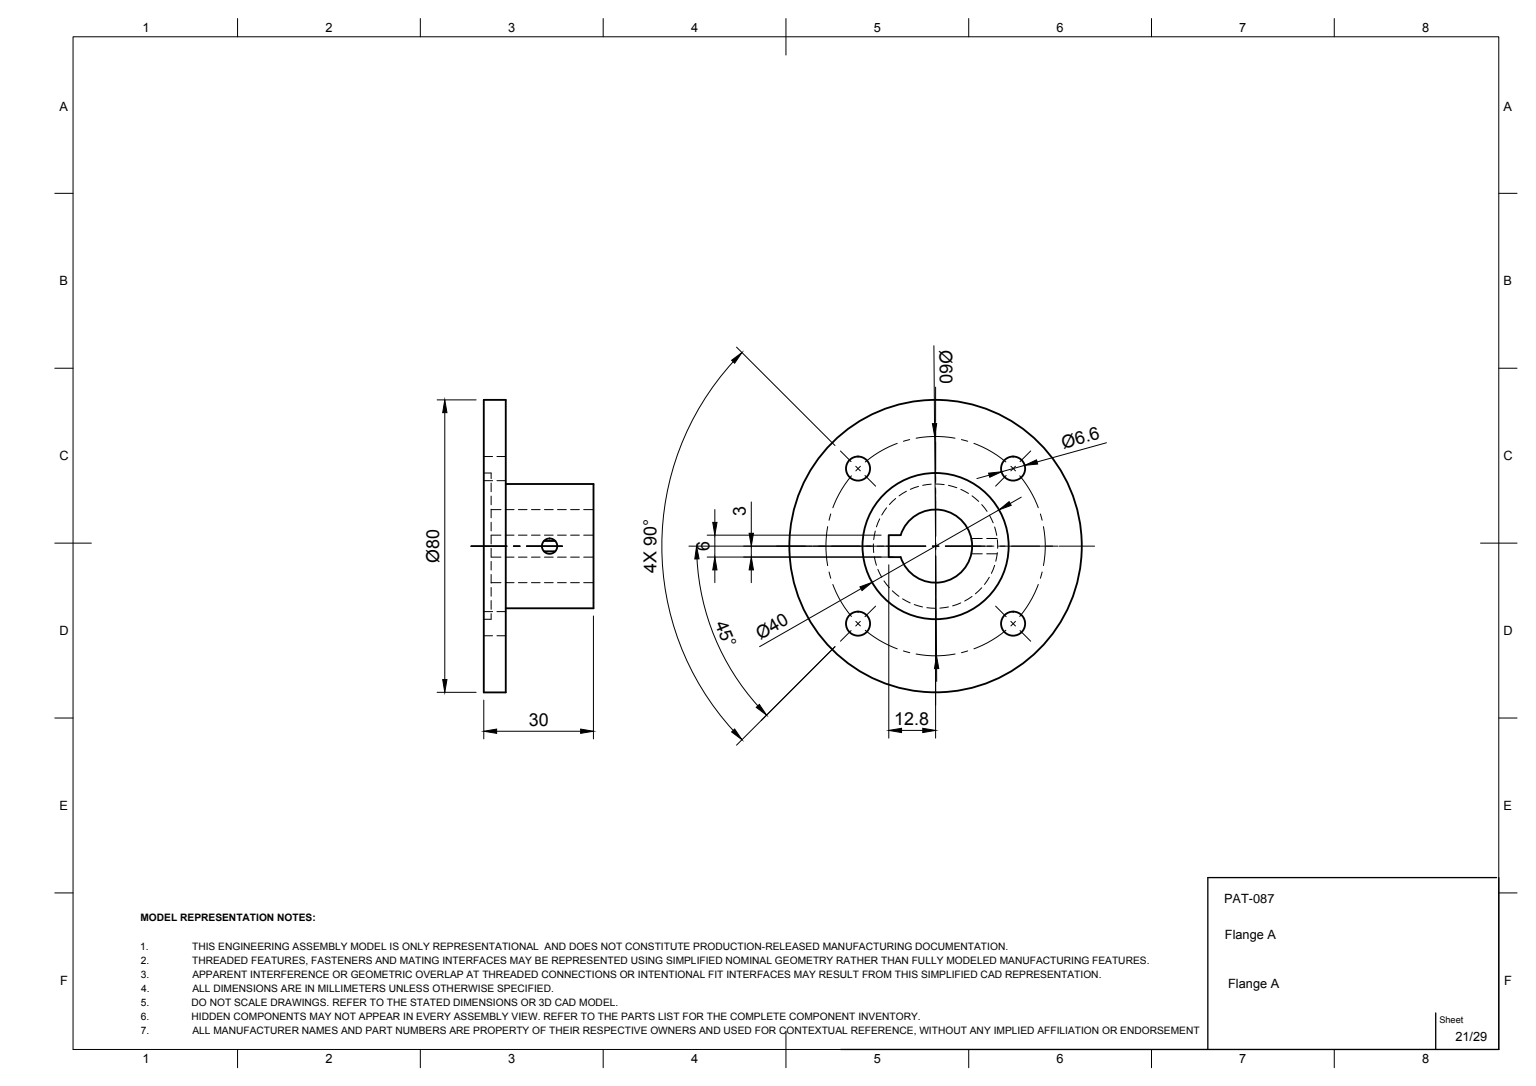
ISO-10303-21;
HEADER;
/* Generated by software containing ST-Developer
 * from STEP Tools, Inc. (www.steptools.com) 
 */

FILE_DESCRIPTION(
/* description */ ('Rigid flange shaft coupling assembly'),
/* implementation_level */ '2;1');

FILE_NAME(
/* name */ 'Flange A.step',
/* time_stamp */ '2026-10-27T10:47:16-07:00',
/* author */ (''),
/* organization */ (''),
/* preprocessor_version */ 'ST-DEVELOPER v20.2',
/* originating_system */ 'Autodesk Translation Framework v15.17.0.0',
/* authorisation */ '');

FILE_SCHEMA (('AUTOMOTIVE_DESIGN { 1 0 10303 214 3 1 1 }'));
ENDSEC;

DATA;
#10=MECHANICAL_DESIGN_GEOMETRIC_PRESENTATION_REPRESENTATION('',(#413),#9141);
#324=B_SPLINE_CURVE_WITH_KNOTS('',3,(#8147,#8148,#8149,#8150,#8151,#8152,
#8153,#8154,#8155,#8156),.UNSPECIFIED.,.F.,.F.,(4,2,2,2,4),(0.803821788694083,
0.87295099185362,0.95230721290097,1.03166343394832,1.10079263710786),
 .UNSPECIFIED.);
#325=B_SPLINE_CURVE_WITH_KNOTS('',3,(#8162,#8163,#8164,#8165,#8166,#8167,
#8168,#8169,#8170,#8171,#8172,#8173,#8174,#8175,#8176,#8177,#8178,#8179),
 .UNSPECIFIED.,.F.,.F.,(4,2,2,2,2,2,2,2,4),(0.,0.0791914196064458,0.158382839212892,
0.237573628052636,0.31676441689238,0.395955205732124,0.475145994571868,
0.554337414178314,0.63352883378476),.UNSPECIFIED.);
#326=B_SPLINE_CURVE_WITH_KNOTS('',3,(#8180,#8181,#8182,#8183,#8184,#8185,
#8186,#8187,#8188,#8189,#8190,#8191,#8192,#8193,#8194,#8195,#8196,#8197),
 .UNSPECIFIED.,.F.,.F.,(4,2,2,2,2,2,2,2,4),(0.63352883378476,0.712720253391205,
0.791911672997651,0.871102461837395,0.95029325067714,1.02948403951688,1.10867482835663,
1.18786624796307,1.26705766756952),.UNSPECIFIED.);
#327=B_SPLINE_CURVE_WITH_KNOTS('',3,(#8200,#8201,#8202,#8203,#8204,#8205,
#8206,#8207,#8208,#8209),.UNSPECIFIED.,.F.,.F.,(4,2,2,2,4),(0.168950313426771,
0.238079516586307,0.317435737633657,0.396791958681006,0.465921161840542),
 .UNSPECIFIED.);
#356=SHAPE_REPRESENTATION_RELATIONSHIP('SRR','None',#9292,#384);
#384=ADVANCED_BREP_SHAPE_REPRESENTATION('',(#441),#9127);
#413=STYLED_ITEM('',(#9493),#441);
#441=MANIFOLD_SOLID_BREP('Body1',#4768);
#519=FACE_BOUND('',#1222,.T.);
#520=FACE_BOUND('',#1225,.T.);
#521=FACE_BOUND('',#1227,.T.);
#522=FACE_BOUND('',#1228,.T.);
#523=FACE_BOUND('',#1229,.T.);
#524=FACE_BOUND('',#1230,.T.);
#525=FACE_BOUND('',#1231,.T.);
#526=FACE_BOUND('',#1234,.T.);
#527=FACE_BOUND('',#1236,.T.);
#528=FACE_BOUND('',#1238,.T.);
#529=FACE_BOUND('',#1239,.T.);
#530=FACE_BOUND('',#1240,.T.);
#531=FACE_BOUND('',#1241,.T.);
#532=FACE_BOUND('',#1242,.T.);
#653=PLANE('',#5338);
#654=PLANE('',#5343);
#655=PLANE('',#5344);
#656=PLANE('',#5345);
#657=PLANE('',#5346);
#658=PLANE('',#5347);
#659=PLANE('',#5353);
#660=PLANE('',#5355);
#661=PLANE('',#5362);
#873=FACE_OUTER_BOUND('',#1211,.T.);
#874=FACE_OUTER_BOUND('',#1212,.T.);
#875=FACE_OUTER_BOUND('',#1213,.T.);
#876=FACE_OUTER_BOUND('',#1214,.T.);
#877=FACE_OUTER_BOUND('',#1215,.T.);
#878=FACE_OUTER_BOUND('',#1216,.T.);
#879=FACE_OUTER_BOUND('',#1217,.T.);
#880=FACE_OUTER_BOUND('',#1218,.T.);
#881=FACE_OUTER_BOUND('',#1219,.T.);
#882=FACE_OUTER_BOUND('',#1220,.T.);
#883=FACE_OUTER_BOUND('',#1221,.T.);
#884=FACE_OUTER_BOUND('',#1223,.T.);
#885=FACE_OUTER_BOUND('',#1224,.T.);
#886=FACE_OUTER_BOUND('',#1226,.T.);
#887=FACE_OUTER_BOUND('',#1232,.T.);
#888=FACE_OUTER_BOUND('',#1233,.T.);
#889=FACE_OUTER_BOUND('',#1235,.T.);
#890=FACE_OUTER_BOUND('',#1237,.T.);
#1211=EDGE_LOOP('',(#3803,#3804,#3805,#3806));
#1212=EDGE_LOOP('',(#3807,#3808,#3809,#3810));
#1213=EDGE_LOOP('',(#3811,#3812,#3813,#3814));
#1214=EDGE_LOOP('',(#3815,#3816,#3817,#3818));
#1215=EDGE_LOOP('',(#3819,#3820));
#1216=EDGE_LOOP('',(#3821,#3822,#3823,#3824,#3825,#3826,#3827,#3828,#3829));
#1217=EDGE_LOOP('',(#3830,#3831,#3832));
#1218=EDGE_LOOP('',(#3833,#3834,#3835,#3836));
#1219=EDGE_LOOP('',(#3837,#3838,#3839,#3840));
#1220=EDGE_LOOP('',(#3841,#3842,#3843,#3844));
#1221=EDGE_LOOP('',(#3845));
#1222=EDGE_LOOP('',(#3846,#3847,#3848,#3849));
#1223=EDGE_LOOP('',(#3850,#3851,#3852,#3853));
#1224=EDGE_LOOP('',(#3854));
#1225=EDGE_LOOP('',(#3855,#3856,#3857,#3858));
#1226=EDGE_LOOP('',(#3859));
#1227=EDGE_LOOP('',(#3860));
#1228=EDGE_LOOP('',(#3861));
#1229=EDGE_LOOP('',(#3862));
#1230=EDGE_LOOP('',(#3863));
#1231=EDGE_LOOP('',(#3864));
#1232=EDGE_LOOP('',(#3865,#3866,#3867,#3868));
#1233=EDGE_LOOP('',(#3869,#3870,#3871,#3872));
#1234=EDGE_LOOP('',(#3873,#3874,#3875,#3876));
#1235=EDGE_LOOP('',(#3877,#3878,#3879,#3880));
#1236=EDGE_LOOP('',(#3881,#3882));
#1237=EDGE_LOOP('',(#3883));
#1238=EDGE_LOOP('',(#3884));
#1239=EDGE_LOOP('',(#3885));
#1240=EDGE_LOOP('',(#3886));
#1241=EDGE_LOOP('',(#3887));
#1242=EDGE_LOOP('',(#3888));
#1578=LINE('',#8120,#1923);
#1579=LINE('',#8126,#1924);
#1580=LINE('',#8132,#1925);
#1581=LINE('',#8138,#1926);
#1582=LINE('',#8143,#1927);
#1583=LINE('',#8160,#1928);
#1584=LINE('',#8211,#1929);
#1585=LINE('',#8215,#1930);
#1586=LINE('',#8217,#1931);
#1587=LINE('',#8219,#1932);
#1588=LINE('',#8220,#1933);
#1589=LINE('',#8223,#1934);
#1590=LINE('',#8225,#1935);
#1591=LINE('',#8226,#1936);
#1592=LINE('',#8229,#1937);
#1593=LINE('',#8231,#1938);
#1594=LINE('',#8232,#1939);
#1595=LINE('',#8241,#1940);
#1596=LINE('',#8253,#1941);
#1597=LINE('',#8256,#1942);
#1923=VECTOR('',#6285,0.33);
#1924=VECTOR('',#6292,0.33);
#1925=VECTOR('',#6299,0.33);
#1926=VECTOR('',#6306,0.33);
#1927=VECTOR('',#6311,1.);
#1928=VECTOR('',#6318,0.21);
#1929=VECTOR('',#6323,1.);
#1930=VECTOR('',#6326,1.);
#1931=VECTOR('',#6327,1.);
#1932=VECTOR('',#6328,1.);
#1933=VECTOR('',#6329,1.);
#1934=VECTOR('',#6332,1.);
#1935=VECTOR('',#6333,1.);
#1936=VECTOR('',#6334,1.);
#1937=VECTOR('',#6337,1.);
#1938=VECTOR('',#6338,1.);
#1939=VECTOR('',#6339,1.);
#1940=VECTOR('',#6350,2.);
#1941=VECTOR('',#6367,4.);
#1942=VECTOR('',#6372,1.7);
#2178=CIRCLE('',#5327,0.33);
#2179=CIRCLE('',#5328,0.33);
#2180=CIRCLE('',#5330,0.33);
#2181=CIRCLE('',#5331,0.33);
#2182=CIRCLE('',#5333,0.33);
#2183=CIRCLE('',#5334,0.33);
#2184=CIRCLE('',#5336,0.33);
#2185=CIRCLE('',#5337,0.33);
#2186=CIRCLE('',#5339,0.21);
#2187=CIRCLE('',#5341,0.21);
#2188=CIRCLE('',#5342,0.21);
#2189=CIRCLE('',#5348,1.7);
#2190=CIRCLE('',#5349,1.);
#2191=CIRCLE('',#5351,2.);
#2192=CIRCLE('',#5352,2.);
#2193=CIRCLE('',#5354,1.);
#2194=CIRCLE('',#5356,4.);
#2195=CIRCLE('',#5357,1.7);
#2196=CIRCLE('',#5359,4.);
#2469=VERTEX_POINT('',#8117);
#2470=VERTEX_POINT('',#8119);
#2471=VERTEX_POINT('',#8123);
#2472=VERTEX_POINT('',#8125);
#2473=VERTEX_POINT('',#8129);
#2474=VERTEX_POINT('',#8131);
#2475=VERTEX_POINT('',#8135);
#2476=VERTEX_POINT('',#8137);
#2477=VERTEX_POINT('',#8141);
#2478=VERTEX_POINT('',#8142);
#2479=VERTEX_POINT('',#8146);
#2480=VERTEX_POINT('',#8157);
#2481=VERTEX_POINT('',#8159);
#2482=VERTEX_POINT('',#8161);
#2483=VERTEX_POINT('',#8198);
#2484=VERTEX_POINT('',#8213);
#2485=VERTEX_POINT('',#8214);
#2486=VERTEX_POINT('',#8216);
#2487=VERTEX_POINT('',#8218);
#2488=VERTEX_POINT('',#8222);
#2489=VERTEX_POINT('',#8224);
#2490=VERTEX_POINT('',#8228);
#2491=VERTEX_POINT('',#8230);
#2492=VERTEX_POINT('',#8234);
#2493=VERTEX_POINT('',#8238);
#2494=VERTEX_POINT('',#8240);
#2495=VERTEX_POINT('',#8246);
#2496=VERTEX_POINT('',#8248);
#2497=VERTEX_POINT('',#8251);
#2945=EDGE_CURVE('',#2469,#2469,#2178,.T.);
#2946=EDGE_CURVE('',#2469,#2470,#1578,.T.);
#2947=EDGE_CURVE('',#2470,#2470,#2179,.T.);
#2948=EDGE_CURVE('',#2471,#2471,#2180,.T.);
#2949=EDGE_CURVE('',#2471,#2472,#1579,.T.);
#2950=EDGE_CURVE('',#2472,#2472,#2181,.T.);
#2951=EDGE_CURVE('',#2473,#2473,#2182,.T.);
#2952=EDGE_CURVE('',#2473,#2474,#1580,.T.);
#2953=EDGE_CURVE('',#2474,#2474,#2183,.T.);
#2954=EDGE_CURVE('',#2475,#2475,#2184,.T.);
#2955=EDGE_CURVE('',#2475,#2476,#1581,.T.);
#2956=EDGE_CURVE('',#2476,#2476,#2185,.T.);
#2957=EDGE_CURVE('',#2477,#2478,#1582,.T.);
#2958=EDGE_CURVE('',#2477,#2478,#2186,.T.);
#2959=EDGE_CURVE('',#2479,#2477,#324,.T.);
#2960=EDGE_CURVE('',#2480,#2479,#2187,.T.);
#2961=EDGE_CURVE('',#2480,#2481,#1583,.T.);
#2962=EDGE_CURVE('',#2482,#2481,#325,.T.);
#2963=EDGE_CURVE('',#2481,#2482,#326,.T.);
#2964=EDGE_CURVE('',#2483,#2480,#2188,.T.);
#2965=EDGE_CURVE('',#2478,#2483,#327,.T.);
#2966=EDGE_CURVE('',#2483,#2479,#1584,.T.);
#2967=EDGE_CURVE('',#2484,#2485,#1585,.T.);
#2968=EDGE_CURVE('',#2484,#2486,#1586,.T.);
#2969=EDGE_CURVE('',#2487,#2486,#1587,.T.);
#2970=EDGE_CURVE('',#2485,#2487,#1588,.T.);
#2971=EDGE_CURVE('',#2488,#2484,#1589,.T.);
#2972=EDGE_CURVE('',#2488,#2489,#1590,.T.);
#2973=EDGE_CURVE('',#2486,#2489,#1591,.T.);
#2974=EDGE_CURVE('',#2490,#2488,#1592,.T.);
#2975=EDGE_CURVE('',#2491,#2490,#1593,.T.);
#2976=EDGE_CURVE('',#2489,#2491,#1594,.T.);
#2977=EDGE_CURVE('',#2492,#2492,#2189,.T.);
#2978=EDGE_CURVE('',#2490,#2485,#2190,.T.);
#2979=EDGE_CURVE('',#2493,#2493,#2191,.T.);
#2980=EDGE_CURVE('',#2493,#2494,#1595,.T.);
#2981=EDGE_CURVE('',#2494,#2494,#2192,.T.);
#2982=EDGE_CURVE('',#2487,#2491,#2193,.T.);
#2983=EDGE_CURVE('',#2495,#2495,#2194,.T.);
#2984=EDGE_CURVE('',#2496,#2496,#2195,.T.);
#2985=EDGE_CURVE('',#2497,#2497,#2196,.T.);
#2986=EDGE_CURVE('',#2497,#2495,#1596,.T.);
#2987=EDGE_CURVE('',#2496,#2492,#1597,.T.);
#3803=ORIENTED_EDGE('',*,*,#2945,.F.);
#3804=ORIENTED_EDGE('',*,*,#2946,.T.);
#3805=ORIENTED_EDGE('',*,*,#2947,.F.);
#3806=ORIENTED_EDGE('',*,*,#2946,.F.);
#3807=ORIENTED_EDGE('',*,*,#2948,.F.);
#3808=ORIENTED_EDGE('',*,*,#2949,.T.);
#3809=ORIENTED_EDGE('',*,*,#2950,.F.);
#3810=ORIENTED_EDGE('',*,*,#2949,.F.);
#3811=ORIENTED_EDGE('',*,*,#2951,.F.);
#3812=ORIENTED_EDGE('',*,*,#2952,.T.);
#3813=ORIENTED_EDGE('',*,*,#2953,.F.);
#3814=ORIENTED_EDGE('',*,*,#2952,.F.);
#3815=ORIENTED_EDGE('',*,*,#2954,.F.);
#3816=ORIENTED_EDGE('',*,*,#2955,.T.);
#3817=ORIENTED_EDGE('',*,*,#2956,.F.);
#3818=ORIENTED_EDGE('',*,*,#2955,.F.);
#3819=ORIENTED_EDGE('',*,*,#2957,.F.);
#3820=ORIENTED_EDGE('',*,*,#2958,.T.);
#3821=ORIENTED_EDGE('',*,*,#2959,.F.);
#3822=ORIENTED_EDGE('',*,*,#2960,.F.);
#3823=ORIENTED_EDGE('',*,*,#2961,.T.);
#3824=ORIENTED_EDGE('',*,*,#2962,.F.);
#3825=ORIENTED_EDGE('',*,*,#2963,.F.);
#3826=ORIENTED_EDGE('',*,*,#2961,.F.);
#3827=ORIENTED_EDGE('',*,*,#2964,.F.);
#3828=ORIENTED_EDGE('',*,*,#2965,.F.);
#3829=ORIENTED_EDGE('',*,*,#2958,.F.);
#3830=ORIENTED_EDGE('',*,*,#2966,.F.);
#3831=ORIENTED_EDGE('',*,*,#2964,.T.);
#3832=ORIENTED_EDGE('',*,*,#2960,.T.);
#3833=ORIENTED_EDGE('',*,*,#2967,.F.);
#3834=ORIENTED_EDGE('',*,*,#2968,.T.);
#3835=ORIENTED_EDGE('',*,*,#2969,.F.);
#3836=ORIENTED_EDGE('',*,*,#2970,.F.);
#3837=ORIENTED_EDGE('',*,*,#2971,.F.);
#3838=ORIENTED_EDGE('',*,*,#2972,.T.);
#3839=ORIENTED_EDGE('',*,*,#2973,.F.);
#3840=ORIENTED_EDGE('',*,*,#2968,.F.);
#3841=ORIENTED_EDGE('',*,*,#2974,.F.);
#3842=ORIENTED_EDGE('',*,*,#2975,.F.);
#3843=ORIENTED_EDGE('',*,*,#2976,.F.);
#3844=ORIENTED_EDGE('',*,*,#2972,.F.);
#3845=ORIENTED_EDGE('',*,*,#2977,.F.);
#3846=ORIENTED_EDGE('',*,*,#2974,.T.);
#3847=ORIENTED_EDGE('',*,*,#2971,.T.);
#3848=ORIENTED_EDGE('',*,*,#2967,.T.);
#3849=ORIENTED_EDGE('',*,*,#2978,.F.);
#3850=ORIENTED_EDGE('',*,*,#2979,.F.);
#3851=ORIENTED_EDGE('',*,*,#2980,.T.);
#3852=ORIENTED_EDGE('',*,*,#2981,.F.);
#3853=ORIENTED_EDGE('',*,*,#2980,.F.);
#3854=ORIENTED_EDGE('',*,*,#2979,.T.);
#3855=ORIENTED_EDGE('',*,*,#2976,.T.);
#3856=ORIENTED_EDGE('',*,*,#2982,.F.);
#3857=ORIENTED_EDGE('',*,*,#2969,.T.);
#3858=ORIENTED_EDGE('',*,*,#2973,.T.);
#3859=ORIENTED_EDGE('',*,*,#2983,.F.);
#3860=ORIENTED_EDGE('',*,*,#2984,.F.);
#3861=ORIENTED_EDGE('',*,*,#2954,.T.);
#3862=ORIENTED_EDGE('',*,*,#2951,.T.);
#3863=ORIENTED_EDGE('',*,*,#2948,.T.);
#3864=ORIENTED_EDGE('',*,*,#2945,.T.);
#3865=ORIENTED_EDGE('',*,*,#2985,.F.);
#3866=ORIENTED_EDGE('',*,*,#2986,.T.);
#3867=ORIENTED_EDGE('',*,*,#2983,.T.);
#3868=ORIENTED_EDGE('',*,*,#2986,.F.);
#3869=ORIENTED_EDGE('',*,*,#2975,.T.);
#3870=ORIENTED_EDGE('',*,*,#2978,.T.);
#3871=ORIENTED_EDGE('',*,*,#2970,.T.);
#3872=ORIENTED_EDGE('',*,*,#2982,.T.);
#3873=ORIENTED_EDGE('',*,*,#2965,.T.);
#3874=ORIENTED_EDGE('',*,*,#2966,.T.);
#3875=ORIENTED_EDGE('',*,*,#2959,.T.);
#3876=ORIENTED_EDGE('',*,*,#2957,.T.);
#3877=ORIENTED_EDGE('',*,*,#2984,.T.);
#3878=ORIENTED_EDGE('',*,*,#2987,.T.);
#3879=ORIENTED_EDGE('',*,*,#2977,.T.);
#3880=ORIENTED_EDGE('',*,*,#2987,.F.);
#3881=ORIENTED_EDGE('',*,*,#2962,.T.);
#3882=ORIENTED_EDGE('',*,*,#2963,.T.);
#3883=ORIENTED_EDGE('',*,*,#2985,.T.);
#3884=ORIENTED_EDGE('',*,*,#2981,.T.);
#3885=ORIENTED_EDGE('',*,*,#2956,.T.);
#3886=ORIENTED_EDGE('',*,*,#2953,.T.);
#3887=ORIENTED_EDGE('',*,*,#2950,.T.);
#3888=ORIENTED_EDGE('',*,*,#2947,.T.);
#4440=CYLINDRICAL_SURFACE('',#5326,0.33);
#4441=CYLINDRICAL_SURFACE('',#5329,0.33);
#4442=CYLINDRICAL_SURFACE('',#5332,0.33);
#4443=CYLINDRICAL_SURFACE('',#5335,0.33);
#4444=CYLINDRICAL_SURFACE('',#5340,0.21);
#4445=CYLINDRICAL_SURFACE('',#5350,2.);
#4446=CYLINDRICAL_SURFACE('',#5358,4.);
#4447=CYLINDRICAL_SURFACE('',#5360,1.);
#4448=CYLINDRICAL_SURFACE('',#5361,1.7);
#4609=ADVANCED_FACE('',(#873),#4440,.F.);
#4610=ADVANCED_FACE('',(#874),#4441,.F.);
#4611=ADVANCED_FACE('',(#875),#4442,.F.);
#4612=ADVANCED_FACE('',(#876),#4443,.F.);
#4613=ADVANCED_FACE('',(#877),#653,.T.);
#4614=ADVANCED_FACE('',(#878),#4444,.F.);
#4615=ADVANCED_FACE('',(#879),#654,.T.);
#4616=ADVANCED_FACE('',(#880),#655,.F.);
#4617=ADVANCED_FACE('',(#881),#656,.F.);
#4618=ADVANCED_FACE('',(#882),#657,.F.);
#4619=ADVANCED_FACE('',(#883,#519),#658,.F.);
#4620=ADVANCED_FACE('',(#884),#4445,.F.);
#4621=ADVANCED_FACE('',(#885,#520),#659,.T.);
#4622=ADVANCED_FACE('',(#886,#521,#522,#523,#524,#525),#660,.F.);
#4623=ADVANCED_FACE('',(#887),#4446,.T.);
#4624=ADVANCED_FACE('',(#888,#526),#4447,.F.);
#4625=ADVANCED_FACE('',(#889,#527),#4448,.T.);
#4626=ADVANCED_FACE('',(#890,#528,#529,#530,#531,#532),#661,.T.);
#4768=CLOSED_SHELL('',(#4609,#4610,#4611,#4612,#4613,#4614,#4615,#4616,
#4617,#4618,#4619,#4620,#4621,#4622,#4623,#4624,#4625,#4626));
#5325=AXIS2_PLACEMENT_3D('',#8115,#6279,#6280);
#5326=AXIS2_PLACEMENT_3D('',#8116,#6281,#6282);
#5327=AXIS2_PLACEMENT_3D('',#8118,#6283,#6284);
#5328=AXIS2_PLACEMENT_3D('',#8121,#6286,#6287);
#5329=AXIS2_PLACEMENT_3D('',#8122,#6288,#6289);
#5330=AXIS2_PLACEMENT_3D('',#8124,#6290,#6291);
#5331=AXIS2_PLACEMENT_3D('',#8127,#6293,#6294);
#5332=AXIS2_PLACEMENT_3D('',#8128,#6295,#6296);
#5333=AXIS2_PLACEMENT_3D('',#8130,#6297,#6298);
#5334=AXIS2_PLACEMENT_3D('',#8133,#6300,#6301);
#5335=AXIS2_PLACEMENT_3D('',#8134,#6302,#6303);
#5336=AXIS2_PLACEMENT_3D('',#8136,#6304,#6305);
#5337=AXIS2_PLACEMENT_3D('',#8139,#6307,#6308);
#5338=AXIS2_PLACEMENT_3D('',#8140,#6309,#6310);
#5339=AXIS2_PLACEMENT_3D('',#8144,#6312,#6313);
#5340=AXIS2_PLACEMENT_3D('',#8145,#6314,#6315);
#5341=AXIS2_PLACEMENT_3D('',#8158,#6316,#6317);
#5342=AXIS2_PLACEMENT_3D('',#8199,#6319,#6320);
#5343=AXIS2_PLACEMENT_3D('',#8210,#6321,#6322);
#5344=AXIS2_PLACEMENT_3D('',#8212,#6324,#6325);
#5345=AXIS2_PLACEMENT_3D('',#8221,#6330,#6331);
#5346=AXIS2_PLACEMENT_3D('',#8227,#6335,#6336);
#5347=AXIS2_PLACEMENT_3D('',#8233,#6340,#6341);
#5348=AXIS2_PLACEMENT_3D('',#8235,#6342,#6343);
#5349=AXIS2_PLACEMENT_3D('',#8236,#6344,#6345);
#5350=AXIS2_PLACEMENT_3D('',#8237,#6346,#6347);
#5351=AXIS2_PLACEMENT_3D('',#8239,#6348,#6349);
#5352=AXIS2_PLACEMENT_3D('',#8242,#6351,#6352);
#5353=AXIS2_PLACEMENT_3D('',#8243,#6353,#6354);
#5354=AXIS2_PLACEMENT_3D('',#8244,#6355,#6356);
#5355=AXIS2_PLACEMENT_3D('',#8245,#6357,#6358);
#5356=AXIS2_PLACEMENT_3D('',#8247,#6359,#6360);
#5357=AXIS2_PLACEMENT_3D('',#8249,#6361,#6362);
#5358=AXIS2_PLACEMENT_3D('',#8250,#6363,#6364);
#5359=AXIS2_PLACEMENT_3D('',#8252,#6365,#6366);
#5360=AXIS2_PLACEMENT_3D('',#8254,#6368,#6369);
#5361=AXIS2_PLACEMENT_3D('',#8255,#6370,#6371);
#5362=AXIS2_PLACEMENT_3D('',#8257,#6373,#6374);
#6279=DIRECTION('axis',(0.,0.,1.));
#6280=DIRECTION('refdir',(1.,0.,0.));
#6281=DIRECTION('center_axis',(0.,1.,0.));
#6282=DIRECTION('ref_axis',(1.,0.,0.));
#6283=DIRECTION('center_axis',(0.,1.,0.));
#6284=DIRECTION('ref_axis',(1.,0.,0.));
#6285=DIRECTION('',(0.,1.,0.));
#6286=DIRECTION('center_axis',(0.,-1.,0.));
#6287=DIRECTION('ref_axis',(1.,0.,0.));
#6288=DIRECTION('center_axis',(0.,1.,0.));
#6289=DIRECTION('ref_axis',(1.,0.,0.));
#6290=DIRECTION('center_axis',(0.,1.,0.));
#6291=DIRECTION('ref_axis',(1.,0.,0.));
#6292=DIRECTION('',(0.,1.,0.));
#6293=DIRECTION('center_axis',(0.,-1.,0.));
#6294=DIRECTION('ref_axis',(1.,0.,0.));
#6295=DIRECTION('center_axis',(0.,1.,0.));
#6296=DIRECTION('ref_axis',(1.,0.,0.));
#6297=DIRECTION('center_axis',(0.,1.,0.));
#6298=DIRECTION('ref_axis',(1.,0.,0.));
#6299=DIRECTION('',(0.,1.,0.));
#6300=DIRECTION('center_axis',(0.,-1.,0.));
#6301=DIRECTION('ref_axis',(1.,0.,0.));
#6302=DIRECTION('center_axis',(0.,1.,0.));
#6303=DIRECTION('ref_axis',(1.,0.,0.));
#6304=DIRECTION('center_axis',(0.,1.,0.));
#6305=DIRECTION('ref_axis',(1.,0.,0.));
#6306=DIRECTION('',(0.,1.,0.));
#6307=DIRECTION('center_axis',(0.,-1.,0.));
#6308=DIRECTION('ref_axis',(1.,0.,0.));
#6309=DIRECTION('center_axis',(0.,0.,1.));
#6310=DIRECTION('ref_axis',(1.,0.,0.));
#6311=DIRECTION('',(0.,1.,0.));
#6312=DIRECTION('center_axis',(0.,0.,1.));
#6313=DIRECTION('ref_axis',(1.,0.,0.));
#6314=DIRECTION('center_axis',(0.,0.,1.));
#6315=DIRECTION('ref_axis',(1.,0.,0.));
#6316=DIRECTION('center_axis',(0.,0.,1.));
#6317=DIRECTION('ref_axis',(1.,0.,0.));
#6318=DIRECTION('',(0.,0.,1.));
#6319=DIRECTION('center_axis',(0.,0.,1.));
#6320=DIRECTION('ref_axis',(1.,0.,0.));
#6321=DIRECTION('center_axis',(0.,0.,1.));
#6322=DIRECTION('ref_axis',(1.,0.,0.));
#6323=DIRECTION('',(0.,-1.,0.));
#6324=DIRECTION('center_axis',(-1.,0.,0.));
#6325=DIRECTION('ref_axis',(0.,0.,1.));
#6326=DIRECTION('',(0.,0.,1.));
#6327=DIRECTION('',(0.,1.,0.));
#6328=DIRECTION('',(0.,0.,-1.));
#6329=DIRECTION('',(0.,1.,0.));
#6330=DIRECTION('center_axis',(0.,0.,-1.));
#6331=DIRECTION('ref_axis',(-1.,0.,0.));
#6332=DIRECTION('',(-1.,0.,0.));
#6333=DIRECTION('',(0.,1.,0.));
#6334=DIRECTION('',(1.,0.,0.));
#6335=DIRECTION('center_axis',(1.,0.,0.));
#6336=DIRECTION('ref_axis',(0.,0.,-1.));
#6337=DIRECTION('',(0.,0.,-1.));
#6338=DIRECTION('',(0.,-1.,0.));
#6339=DIRECTION('',(0.,0.,1.));
#6340=DIRECTION('center_axis',(0.,1.,0.));
#6341=DIRECTION('ref_axis',(1.,0.,0.));
#6342=DIRECTION('center_axis',(0.,1.,0.));
#6343=DIRECTION('ref_axis',(1.,0.,0.));
#6344=DIRECTION('center_axis',(0.,-1.,0.));
#6345=DIRECTION('ref_axis',(1.,0.,0.));
#6346=DIRECTION('center_axis',(0.,1.,0.));
#6347=DIRECTION('ref_axis',(1.,0.,0.));
#6348=DIRECTION('center_axis',(0.,1.,0.));
#6349=DIRECTION('ref_axis',(1.,0.,0.));
#6350=DIRECTION('',(0.,1.,0.));
#6351=DIRECTION('center_axis',(0.,-1.,0.));
#6352=DIRECTION('ref_axis',(1.,0.,0.));
#6353=DIRECTION('center_axis',(0.,1.,0.));
#6354=DIRECTION('ref_axis',(1.,0.,0.));
#6355=DIRECTION('center_axis',(0.,1.,0.));
#6356=DIRECTION('ref_axis',(1.,0.,0.));
#6357=DIRECTION('center_axis',(0.,1.,0.));
#6358=DIRECTION('ref_axis',(1.,0.,0.));
#6359=DIRECTION('center_axis',(0.,1.,0.));
#6360=DIRECTION('ref_axis',(1.,0.,0.));
#6361=DIRECTION('center_axis',(0.,-1.,0.));
#6362=DIRECTION('ref_axis',(1.,0.,0.));
#6363=DIRECTION('center_axis',(0.,1.,0.));
#6364=DIRECTION('ref_axis',(1.,0.,0.));
#6365=DIRECTION('center_axis',(0.,1.,0.));
#6366=DIRECTION('ref_axis',(1.,0.,0.));
#6367=DIRECTION('',(0.,-1.,0.));
#6368=DIRECTION('center_axis',(0.,1.,0.));
#6369=DIRECTION('ref_axis',(6.12323399573677E-17,0.,1.));
#6370=DIRECTION('center_axis',(0.,1.,0.));
#6371=DIRECTION('ref_axis',(1.,0.,0.));
#6372=DIRECTION('',(0.,-1.,0.));
#6373=DIRECTION('center_axis',(0.,1.,0.));
#6374=DIRECTION('ref_axis',(1.,0.,0.));
#8115=CARTESIAN_POINT('',(0.,0.,0.));
#8116=CARTESIAN_POINT('Origin',(-2.12132034355964,9.3,4.40867965644036));
#8117=CARTESIAN_POINT('',(-2.45132034355964,9.4,4.40867965644036));
#8118=CARTESIAN_POINT('Origin',(-2.12132034355964,9.4,4.40867965644036));
#8119=CARTESIAN_POINT('',(-2.45132034355964,10.,4.40867965644036));
#8120=CARTESIAN_POINT('',(-2.45132034355964,9.3,4.40867965644036));
#8121=CARTESIAN_POINT('Origin',(-2.12132034355964,10.,4.40867965644036));
#8122=CARTESIAN_POINT('Origin',(-2.12132034355964,9.3,8.65132034355964));
#8123=CARTESIAN_POINT('',(-2.45132034355964,9.4,8.65132034355964));
#8124=CARTESIAN_POINT('Origin',(-2.12132034355964,9.4,8.65132034355964));
#8125=CARTESIAN_POINT('',(-2.45132034355964,10.,8.65132034355964));
#8126=CARTESIAN_POINT('',(-2.45132034355964,9.3,8.65132034355964));
#8127=CARTESIAN_POINT('Origin',(-2.12132034355964,10.,8.65132034355964));
#8128=CARTESIAN_POINT('Origin',(2.12132034355964,9.3,8.65132034355964));
#8129=CARTESIAN_POINT('',(1.79132034355964,9.4,8.65132034355964));
#8130=CARTESIAN_POINT('Origin',(2.12132034355964,9.4,8.65132034355964));
#8131=CARTESIAN_POINT('',(1.79132034355964,10.,8.65132034355964));
#8132=CARTESIAN_POINT('',(1.79132034355964,9.3,8.65132034355964));
#8133=CARTESIAN_POINT('Origin',(2.12132034355964,10.,8.65132034355964));
#8134=CARTESIAN_POINT('Origin',(2.12132034355964,9.3,4.40867965644036));
#8135=CARTESIAN_POINT('',(1.79132034355964,9.4,4.40867965644036));
#8136=CARTESIAN_POINT('Origin',(2.12132034355964,9.4,4.40867965644036));
#8137=CARTESIAN_POINT('',(1.79132034355964,10.,4.40867965644036));
#8138=CARTESIAN_POINT('',(1.79132034355964,9.3,4.40867965644036));
#8139=CARTESIAN_POINT('Origin',(2.12132034355964,10.,4.40867965644036));
#8140=CARTESIAN_POINT('Origin',(0.,8.2,7.52));
#8141=CARTESIAN_POINT('',(0.141067359796651,8.04443650813895,7.52));
#8142=CARTESIAN_POINT('',(0.141067359796651,8.35556349186105,7.52));
#8143=CARTESIAN_POINT('',(0.141067359796651,7.,7.52));
#8144=CARTESIAN_POINT('Origin',(0.,8.2,7.52));
#8145=CARTESIAN_POINT('Origin',(0.,8.2,7.52));
#8146=CARTESIAN_POINT('',(-0.141067359796651,8.04443650813895,7.52));
#8147=CARTESIAN_POINT('Ctrl Pts',(-0.141067359796651,8.04443650813895,7.52));
#8148=CARTESIAN_POINT('Ctrl Pts',(-0.123818356698219,8.0287948476368,7.52245784982447));
#8149=CARTESIAN_POINT('Ctrl Pts',(-0.102998643109696,8.01537595666898,7.52493819304946));
#8150=CARTESIAN_POINT('Ctrl Pts',(-0.0546141143983529,7.99530253627557,
7.52884449237241));
#8151=CARTESIAN_POINT('Ctrl Pts',(-0.0264520736824499,7.99,7.53));
#8152=CARTESIAN_POINT('Ctrl Pts',(0.0264520736824498,7.99,7.53));
#8153=CARTESIAN_POINT('Ctrl Pts',(0.0546141143983527,7.99530253627557,7.52884449237241));
#8154=CARTESIAN_POINT('Ctrl Pts',(0.102998643109696,8.01537595666898,7.52493819304946));
#8155=CARTESIAN_POINT('Ctrl Pts',(0.123818356698219,8.0287948476368,7.52245784982447));
#8156=CARTESIAN_POINT('Ctrl Pts',(0.141067359796651,8.04443650813895,7.52));
#8157=CARTESIAN_POINT('',(-0.21,8.2,7.52));
#8158=CARTESIAN_POINT('Origin',(0.,8.2,7.52));
#8159=CARTESIAN_POINT('',(-0.21,8.2,8.21697954937219));
#8160=CARTESIAN_POINT('',(-0.21,8.2,7.52));
#8161=CARTESIAN_POINT('',(0.21,8.2,8.21697954937219));
#8162=CARTESIAN_POINT('Ctrl Pts',(0.21,8.2,8.21697954937219));
#8163=CARTESIAN_POINT('Ctrl Pts',(0.21,8.17360286013118,8.21697954937219));
#8164=CARTESIAN_POINT('Ctrl Pts',(0.204718998643499,8.14546483574125,8.21766304765575));
#8165=CARTESIAN_POINT('Ctrl Pts',(0.183279390356407,8.09373326708872,8.22012576310987));
#8166=CARTESIAN_POINT('Ctrl Pts',(0.167122246533942,8.07013739843559,8.22186875774124));
#8167=CARTESIAN_POINT('Ctrl Pts',(0.129862749952602,8.03287790185425,8.22513580556568));
#8168=CARTESIAN_POINT('Ctrl Pts',(0.106266816759542,8.0167206417943,8.22687297932906));
#8169=CARTESIAN_POINT('Ctrl Pts',(0.0545350296960238,7.99528094818772,8.22932235754078));
#8170=CARTESIAN_POINT('Ctrl Pts',(0.026396929613248,7.99,8.23));
#8171=CARTESIAN_POINT('Ctrl Pts',(-0.026396929613248,7.99,8.23));
#8172=CARTESIAN_POINT('Ctrl Pts',(-0.0545350296960238,7.99528094818772,
8.22932235754078));
#8173=CARTESIAN_POINT('Ctrl Pts',(-0.106266816759542,8.0167206417943,8.22687297932906));
#8174=CARTESIAN_POINT('Ctrl Pts',(-0.129862749952602,8.03287790185425,8.22513580556568));
#8175=CARTESIAN_POINT('Ctrl Pts',(-0.167122246533942,8.07013739843559,8.22186875774124));
#8176=CARTESIAN_POINT('Ctrl Pts',(-0.183279390356407,8.09373326708872,8.22012576310987));
#8177=CARTESIAN_POINT('Ctrl Pts',(-0.204718998643499,8.14546483574125,8.21766304765575));
#8178=CARTESIAN_POINT('Ctrl Pts',(-0.21,8.17360286013118,8.21697954937219));
#8179=CARTESIAN_POINT('Ctrl Pts',(-0.21,8.2,8.21697954937219));
#8180=CARTESIAN_POINT('Ctrl Pts',(-0.21,8.2,8.21697954937219));
#8181=CARTESIAN_POINT('Ctrl Pts',(-0.21,8.22639713986882,8.21697954937219));
#8182=CARTESIAN_POINT('Ctrl Pts',(-0.204718998643499,8.25453516425875,8.21766304765575));
#8183=CARTESIAN_POINT('Ctrl Pts',(-0.183279390356407,8.30626673291128,8.22012576310987));
#8184=CARTESIAN_POINT('Ctrl Pts',(-0.167122246533942,8.32986260156441,8.22186875774124));
#8185=CARTESIAN_POINT('Ctrl Pts',(-0.129862749952602,8.36712209814575,8.22513580556568));
#8186=CARTESIAN_POINT('Ctrl Pts',(-0.106266816759542,8.3832793582057,8.22687297932906));
#8187=CARTESIAN_POINT('Ctrl Pts',(-0.0545350296960238,8.40471905181228,
8.22932235754078));
#8188=CARTESIAN_POINT('Ctrl Pts',(-0.0263969296132481,8.41,8.23));
#8189=CARTESIAN_POINT('Ctrl Pts',(0.026396929613248,8.41,8.23));
#8190=CARTESIAN_POINT('Ctrl Pts',(0.0545350296960237,8.40471905181228,8.22932235754078));
#8191=CARTESIAN_POINT('Ctrl Pts',(0.106266816759542,8.3832793582057,8.22687297932906));
#8192=CARTESIAN_POINT('Ctrl Pts',(0.129862749952602,8.36712209814575,8.22513580556568));
#8193=CARTESIAN_POINT('Ctrl Pts',(0.167122246533941,8.32986260156441,8.22186875774124));
#8194=CARTESIAN_POINT('Ctrl Pts',(0.183279390356407,8.30626673291128,8.22012576310987));
#8195=CARTESIAN_POINT('Ctrl Pts',(0.204718998643499,8.25453516425875,8.21766304765575));
#8196=CARTESIAN_POINT('Ctrl Pts',(0.21,8.22639713986882,8.21697954937219));
#8197=CARTESIAN_POINT('Ctrl Pts',(0.21,8.2,8.21697954937219));
#8198=CARTESIAN_POINT('',(-0.141067359796651,8.35556349186105,7.52));
#8199=CARTESIAN_POINT('Origin',(0.,8.2,7.52));
#8200=CARTESIAN_POINT('Ctrl Pts',(0.14106735979665,8.35556349186105,7.52));
#8201=CARTESIAN_POINT('Ctrl Pts',(0.123818356698217,8.3712051523632,7.52245784982447));
#8202=CARTESIAN_POINT('Ctrl Pts',(0.102998643109696,8.38462404333102,7.52493819304946));
#8203=CARTESIAN_POINT('Ctrl Pts',(0.0546141143983528,8.40469746372443,7.52884449237241));
#8204=CARTESIAN_POINT('Ctrl Pts',(0.0264520736824499,8.41,7.53));
#8205=CARTESIAN_POINT('Ctrl Pts',(-0.0264520736824498,8.41,7.53));
#8206=CARTESIAN_POINT('Ctrl Pts',(-0.0546141143983528,8.40469746372443,
7.52884449237241));
#8207=CARTESIAN_POINT('Ctrl Pts',(-0.102998643109695,8.38462404333102,7.52493819304946));
#8208=CARTESIAN_POINT('Ctrl Pts',(-0.123818356698218,8.3712051523632,7.52245784982447));
#8209=CARTESIAN_POINT('Ctrl Pts',(-0.14106735979665,8.35556349186105,7.52));
#8210=CARTESIAN_POINT('Origin',(0.,8.2,7.52));
#8211=CARTESIAN_POINT('',(-0.141067359796651,7.,7.52));
#8212=CARTESIAN_POINT('Origin',(-0.3,6.9,5.25));
#8213=CARTESIAN_POINT('',(-0.3,7.,5.25));
#8214=CARTESIAN_POINT('',(-0.3,7.,5.57606079858305));
#8215=CARTESIAN_POINT('',(-0.3,7.,5.89));
#8216=CARTESIAN_POINT('',(-0.3,9.8,5.25));
#8217=CARTESIAN_POINT('',(-0.3,6.9,5.25));
#8218=CARTESIAN_POINT('',(-0.3,9.8,5.57606079858305));
#8219=CARTESIAN_POINT('',(-0.3,9.8,5.89));
#8220=CARTESIAN_POINT('',(-0.3,7.,5.57606079858305));
#8221=CARTESIAN_POINT('Origin',(0.3,6.9,5.25));
#8222=CARTESIAN_POINT('',(0.3,7.,5.25));
#8223=CARTESIAN_POINT('',(0.15,7.,5.25));
#8224=CARTESIAN_POINT('',(0.3,9.8,5.25));
#8225=CARTESIAN_POINT('',(0.3,6.9,5.25));
#8226=CARTESIAN_POINT('',(0.15,9.8,5.25));
#8227=CARTESIAN_POINT('Origin',(0.3,6.9,6.53));
#8228=CARTESIAN_POINT('',(0.3,7.,5.57606079858305));
#8229=CARTESIAN_POINT('',(0.3,7.,6.53));
#8230=CARTESIAN_POINT('',(0.3,9.8,5.57606079858305));
#8231=CARTESIAN_POINT('',(0.3,7.,5.57606079858305));
#8232=CARTESIAN_POINT('',(0.3,9.8,6.53));
#8233=CARTESIAN_POINT('Origin',(0.,7.,6.53));
#8234=CARTESIAN_POINT('',(-1.7,7.,6.53));
#8235=CARTESIAN_POINT('Origin',(0.,7.,6.53));
#8236=CARTESIAN_POINT('Origin',(0.,7.,6.53));
#8237=CARTESIAN_POINT('Origin',(0.,9.8,6.53));
#8238=CARTESIAN_POINT('',(-2.,9.8,6.53));
#8239=CARTESIAN_POINT('Origin',(0.,9.8,6.53));
#8240=CARTESIAN_POINT('',(-2.,10.,6.53));
#8241=CARTESIAN_POINT('',(-2.,9.8,6.53));
#8242=CARTESIAN_POINT('Origin',(0.,10.,6.53));
#8243=CARTESIAN_POINT('Origin',(0.,9.8,6.53));
#8244=CARTESIAN_POINT('Origin',(0.,9.8,6.53));
#8245=CARTESIAN_POINT('Origin',(0.,9.4,6.53));
#8246=CARTESIAN_POINT('',(-4.,9.4,6.53));
#8247=CARTESIAN_POINT('Origin',(0.,9.4,6.53));
#8248=CARTESIAN_POINT('',(-1.7,9.4,6.53));
#8249=CARTESIAN_POINT('Origin',(0.,9.4,6.53));
#8250=CARTESIAN_POINT('Origin',(0.,9.4,6.53));
#8251=CARTESIAN_POINT('',(-4.,10.,6.53));
#8252=CARTESIAN_POINT('Origin',(0.,10.,6.53));
#8253=CARTESIAN_POINT('',(-4.,9.4,6.53));
#8254=CARTESIAN_POINT('Origin',(0.,7.,6.53));
#8255=CARTESIAN_POINT('Origin',(0.,7.,6.53));
#8256=CARTESIAN_POINT('',(-1.7,7.,6.53));
#8257=CARTESIAN_POINT('Origin',(0.,10.,6.53));
#9094=UNCERTAINTY_MEASURE_WITH_UNIT(LENGTH_MEASURE(0.001),#9142,
'DISTANCE_ACCURACY_VALUE',
'Maximum model space distance between geometric entities at asserted c
onnectivities');
#9108=UNCERTAINTY_MEASURE_WITH_UNIT(LENGTH_MEASURE(0.001),#9142,
'DISTANCE_ACCURACY_VALUE',
'Maximum model space distance between geometric entities at asserted c
onnectivities');
#9127=(
GEOMETRIC_REPRESENTATION_CONTEXT(3)
GLOBAL_UNCERTAINTY_ASSIGNED_CONTEXT((#9094))
GLOBAL_UNIT_ASSIGNED_CONTEXT((#9142,#9144,#9145))
REPRESENTATION_CONTEXT('','3D')
);
#9141=(
GEOMETRIC_REPRESENTATION_CONTEXT(3)
GLOBAL_UNCERTAINTY_ASSIGNED_CONTEXT((#9108))
GLOBAL_UNIT_ASSIGNED_CONTEXT((#9142,#9144,#9145))
REPRESENTATION_CONTEXT('','3D')
);
#9142=(
LENGTH_UNIT()
NAMED_UNIT(*)
SI_UNIT(.CENTI.,.METRE.)
);
#9144=(
NAMED_UNIT(*)
PLANE_ANGLE_UNIT()
SI_UNIT($,.RADIAN.)
);
#9145=(
NAMED_UNIT(*)
SI_UNIT($,.STERADIAN.)
SOLID_ANGLE_UNIT()
);
#9164=SHAPE_DEFINITION_REPRESENTATION(#9198,#9292);
#9198=PRODUCT_DEFINITION_SHAPE('',$,#9325);
#9292=SHAPE_REPRESENTATION('',(#5325),#9127);
#9306=PRODUCT_DEFINITION_CONTEXT('part definition',#9404,'design');
#9325=PRODUCT_DEFINITION('Flange A','Flange A',#9357,#9306);
#9357=PRODUCT_DEFINITION_FORMATION('',$,#9424);
#9404=APPLICATION_CONTEXT(
'Core Data for Automotive Mechanical Design Process');
#9405=PRODUCT_CONTEXT('part definition',#9404,'mechanical');
#9424=PRODUCT('Flange A','Flange A','Flange A',(#9405));
#9487=COLOUR_RGB('Sky Blue',0.24,0.69,0.87);
#9488=FILL_AREA_STYLE_COLOUR('',#9487);
#9489=FILL_AREA_STYLE('',(#9488));
#9490=SURFACE_STYLE_FILL_AREA(#9489);
#9491=SURFACE_SIDE_STYLE('',(#9490));
#9492=SURFACE_STYLE_USAGE(.BOTH.,#9491);
#9493=PRESENTATION_STYLE_ASSIGNMENT((#9492));
ENDSEC;
END-ISO-10303-21;
